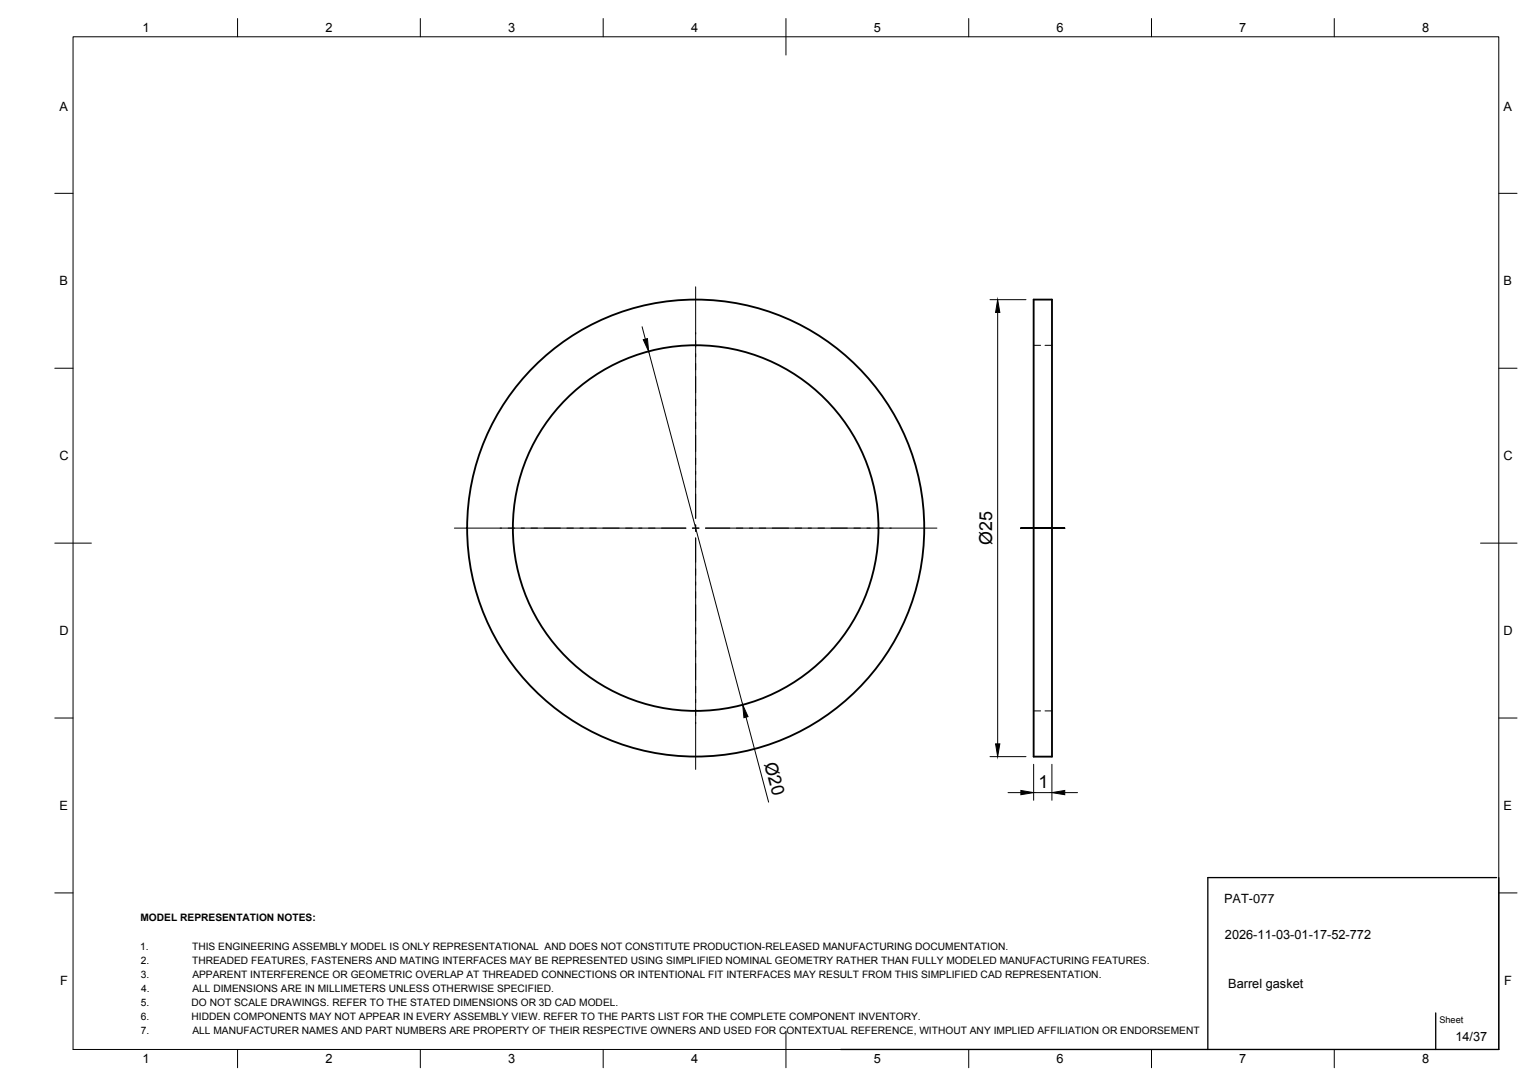
ISO-10303-21;
HEADER;
/* Generated by software containing ST-Developer
 * from STEP Tools, Inc. (www.steptools.com) 
 */

FILE_DESCRIPTION(
/* description */ ('Pallet stop with pneumatic fitting'),
/* implementation_level */ '2;1');

FILE_NAME(
/* name */ 'Barrel gasket.step',
/* time_stamp */ '2026-10-27T10:51:41-07:00',
/* author */ (''),
/* organization */ (''),
/* preprocessor_version */ 'ST-DEVELOPER v20.2',
/* originating_system */ 'Autodesk Translation Framework v15.17.0.0',
/* authorisation */ '');

FILE_SCHEMA (('AUTOMOTIVE_DESIGN { 1 0 10303 214 3 1 1 }'));
ENDSEC;

DATA;
#10=MECHANICAL_DESIGN_GEOMETRIC_PRESENTATION_REPRESENTATION('',(#366),#10265);
#302=SHAPE_REPRESENTATION_RELATIONSHIP('SRR','None',#10415,#334);
#334=ADVANCED_BREP_SHAPE_REPRESENTATION('',(#398),#10239);
#366=STYLED_ITEM('',(#10641),#398);
#398=MANIFOLD_SOLID_BREP('Body1',#5054);
#478=FACE_BOUND('',#1218,.T.);
#479=FACE_BOUND('',#1220,.T.);
#606=PLANE('',#5645);
#607=PLANE('',#5646);
#842=FACE_OUTER_BOUND('',#1215,.T.);
#843=FACE_OUTER_BOUND('',#1216,.T.);
#844=FACE_OUTER_BOUND('',#1217,.T.);
#845=FACE_OUTER_BOUND('',#1219,.T.);
#1215=EDGE_LOOP('',(#3832,#3833,#3834,#3835));
#1216=EDGE_LOOP('',(#3836,#3837,#3838,#3839));
#1217=EDGE_LOOP('',(#3840));
#1218=EDGE_LOOP('',(#3841));
#1219=EDGE_LOOP('',(#3842));
#1220=EDGE_LOOP('',(#3843));
#1607=LINE('',#9095,#1942);
#1608=LINE('',#9101,#1943);
#1942=VECTOR('',#6624,1.);
#1943=VECTOR('',#6631,1.25);
#2250=CIRCLE('',#5640,1.);
#2251=CIRCLE('',#5641,1.);
#2252=CIRCLE('',#5643,1.25);
#2253=CIRCLE('',#5644,1.25);
#2546=VERTEX_POINT('',#9092);
#2547=VERTEX_POINT('',#9094);
#2548=VERTEX_POINT('',#9098);
#2549=VERTEX_POINT('',#9100);
#3015=EDGE_CURVE('',#2546,#2546,#2250,.T.);
#3016=EDGE_CURVE('',#2546,#2547,#1607,.T.);
#3017=EDGE_CURVE('',#2547,#2547,#2251,.T.);
#3018=EDGE_CURVE('',#2548,#2548,#2252,.T.);
#3019=EDGE_CURVE('',#2548,#2549,#1608,.T.);
#3020=EDGE_CURVE('',#2549,#2549,#2253,.T.);
#3832=ORIENTED_EDGE('',*,*,#3015,.F.);
#3833=ORIENTED_EDGE('',*,*,#3016,.T.);
#3834=ORIENTED_EDGE('',*,*,#3017,.T.);
#3835=ORIENTED_EDGE('',*,*,#3016,.F.);
#3836=ORIENTED_EDGE('',*,*,#3018,.F.);
#3837=ORIENTED_EDGE('',*,*,#3019,.T.);
#3838=ORIENTED_EDGE('',*,*,#3020,.T.);
#3839=ORIENTED_EDGE('',*,*,#3019,.F.);
#3840=ORIENTED_EDGE('',*,*,#3018,.T.);
#3841=ORIENTED_EDGE('',*,*,#3015,.T.);
#3842=ORIENTED_EDGE('',*,*,#3020,.F.);
#3843=ORIENTED_EDGE('',*,*,#3017,.F.);
#4666=CYLINDRICAL_SURFACE('',#5639,1.);
#4667=CYLINDRICAL_SURFACE('',#5642,1.25);
#4837=ADVANCED_FACE('',(#842),#4666,.F.);
#4838=ADVANCED_FACE('',(#843),#4667,.T.);
#4839=ADVANCED_FACE('',(#844,#478),#606,.T.);
#4840=ADVANCED_FACE('',(#845,#479),#607,.F.);
#5054=CLOSED_SHELL('',(#4837,#4838,#4839,#4840));
#5638=AXIS2_PLACEMENT_3D('',#9090,#6618,#6619);
#5639=AXIS2_PLACEMENT_3D('',#9091,#6620,#6621);
#5640=AXIS2_PLACEMENT_3D('',#9093,#6622,#6623);
#5641=AXIS2_PLACEMENT_3D('',#9096,#6625,#6626);
#5642=AXIS2_PLACEMENT_3D('',#9097,#6627,#6628);
#5643=AXIS2_PLACEMENT_3D('',#9099,#6629,#6630);
#5644=AXIS2_PLACEMENT_3D('',#9102,#6632,#6633);
#5645=AXIS2_PLACEMENT_3D('',#9103,#6634,#6635);
#5646=AXIS2_PLACEMENT_3D('',#9104,#6636,#6637);
#6618=DIRECTION('axis',(0.,0.,1.));
#6619=DIRECTION('refdir',(1.,0.,0.));
#6620=DIRECTION('center_axis',(0.,0.,1.));
#6621=DIRECTION('ref_axis',(1.,0.,0.));
#6622=DIRECTION('center_axis',(0.,0.,-1.));
#6623=DIRECTION('ref_axis',(1.,0.,0.));
#6624=DIRECTION('',(0.,0.,-1.));
#6625=DIRECTION('center_axis',(0.,0.,-1.));
#6626=DIRECTION('ref_axis',(1.,0.,0.));
#6627=DIRECTION('center_axis',(0.,0.,1.));
#6628=DIRECTION('ref_axis',(1.,0.,0.));
#6629=DIRECTION('center_axis',(0.,0.,1.));
#6630=DIRECTION('ref_axis',(1.,0.,0.));
#6631=DIRECTION('',(0.,0.,-1.));
#6632=DIRECTION('center_axis',(0.,0.,1.));
#6633=DIRECTION('ref_axis',(1.,0.,0.));
#6634=DIRECTION('center_axis',(0.,0.,1.));
#6635=DIRECTION('ref_axis',(1.,0.,0.));
#6636=DIRECTION('center_axis',(0.,0.,1.));
#6637=DIRECTION('ref_axis',(1.,0.,0.));
#9090=CARTESIAN_POINT('',(0.,0.,0.));
#9091=CARTESIAN_POINT('Origin',(4.,4.,1.9));
#9092=CARTESIAN_POINT('',(3.,4.,2.));
#9093=CARTESIAN_POINT('Origin',(4.,4.,2.));
#9094=CARTESIAN_POINT('',(3.,4.,1.9));
#9095=CARTESIAN_POINT('',(3.,4.,1.9));
#9096=CARTESIAN_POINT('Origin',(4.,4.,1.9));
#9097=CARTESIAN_POINT('Origin',(4.,4.,1.9));
#9098=CARTESIAN_POINT('',(2.75,4.,2.));
#9099=CARTESIAN_POINT('Origin',(4.,4.,2.));
#9100=CARTESIAN_POINT('',(2.75,4.,1.9));
#9101=CARTESIAN_POINT('',(2.75,4.,1.9));
#9102=CARTESIAN_POINT('Origin',(4.,4.,1.9));
#9103=CARTESIAN_POINT('Origin',(4.,4.,2.));
#9104=CARTESIAN_POINT('Origin',(4.,4.,1.9));
#10201=UNCERTAINTY_MEASURE_WITH_UNIT(LENGTH_MEASURE(0.001),#10266,
'DISTANCE_ACCURACY_VALUE',
'Maximum model space distance between geometric entities at asserted c
onnectivities');
#10227=UNCERTAINTY_MEASURE_WITH_UNIT(LENGTH_MEASURE(0.001),#10266,
'DISTANCE_ACCURACY_VALUE',
'Maximum model space distance between geometric entities at asserted c
onnectivities');
#10239=(
GEOMETRIC_REPRESENTATION_CONTEXT(3)
GLOBAL_UNCERTAINTY_ASSIGNED_CONTEXT((#10201))
GLOBAL_UNIT_ASSIGNED_CONTEXT((#10266,#10268,#10269))
REPRESENTATION_CONTEXT('','3D')
);
#10265=(
GEOMETRIC_REPRESENTATION_CONTEXT(3)
GLOBAL_UNCERTAINTY_ASSIGNED_CONTEXT((#10227))
GLOBAL_UNIT_ASSIGNED_CONTEXT((#10266,#10268,#10269))
REPRESENTATION_CONTEXT('','3D')
);
#10266=(
LENGTH_UNIT()
NAMED_UNIT(*)
SI_UNIT(.CENTI.,.METRE.)
);
#10268=(
NAMED_UNIT(*)
PLANE_ANGLE_UNIT()
SI_UNIT($,.RADIAN.)
);
#10269=(
NAMED_UNIT(*)
SI_UNIT($,.STERADIAN.)
SOLID_ANGLE_UNIT()
);
#10281=SHAPE_DEFINITION_REPRESENTATION(#10318,#10415);
#10318=PRODUCT_DEFINITION_SHAPE('',$,#10453);
#10415=SHAPE_REPRESENTATION('',(#5638),#10239);
#10441=PRODUCT_DEFINITION_CONTEXT('part definition',#10554,'design');
#10453=PRODUCT_DEFINITION('Barrel gasket','Barrel gasket',#10490,#10441);
#10490=PRODUCT_DEFINITION_FORMATION('',$,#10567);
#10554=APPLICATION_CONTEXT(
'Core Data for Automotive Mechanical Design Process');
#10555=PRODUCT_CONTEXT('part definition',#10554,'mechanical');
#10567=PRODUCT('Barrel gasket','Barrel gasket','Barrel gasket',(#10555));
#10635=COLOUR_RGB('Light Blue',0.38,0.62,0.78);
#10636=FILL_AREA_STYLE_COLOUR('',#10635);
#10637=FILL_AREA_STYLE('',(#10636));
#10638=SURFACE_STYLE_FILL_AREA(#10637);
#10639=SURFACE_SIDE_STYLE('',(#10638));
#10640=SURFACE_STYLE_USAGE(.BOTH.,#10639);
#10641=PRESENTATION_STYLE_ASSIGNMENT((#10640));
ENDSEC;
END-ISO-10303-21;
